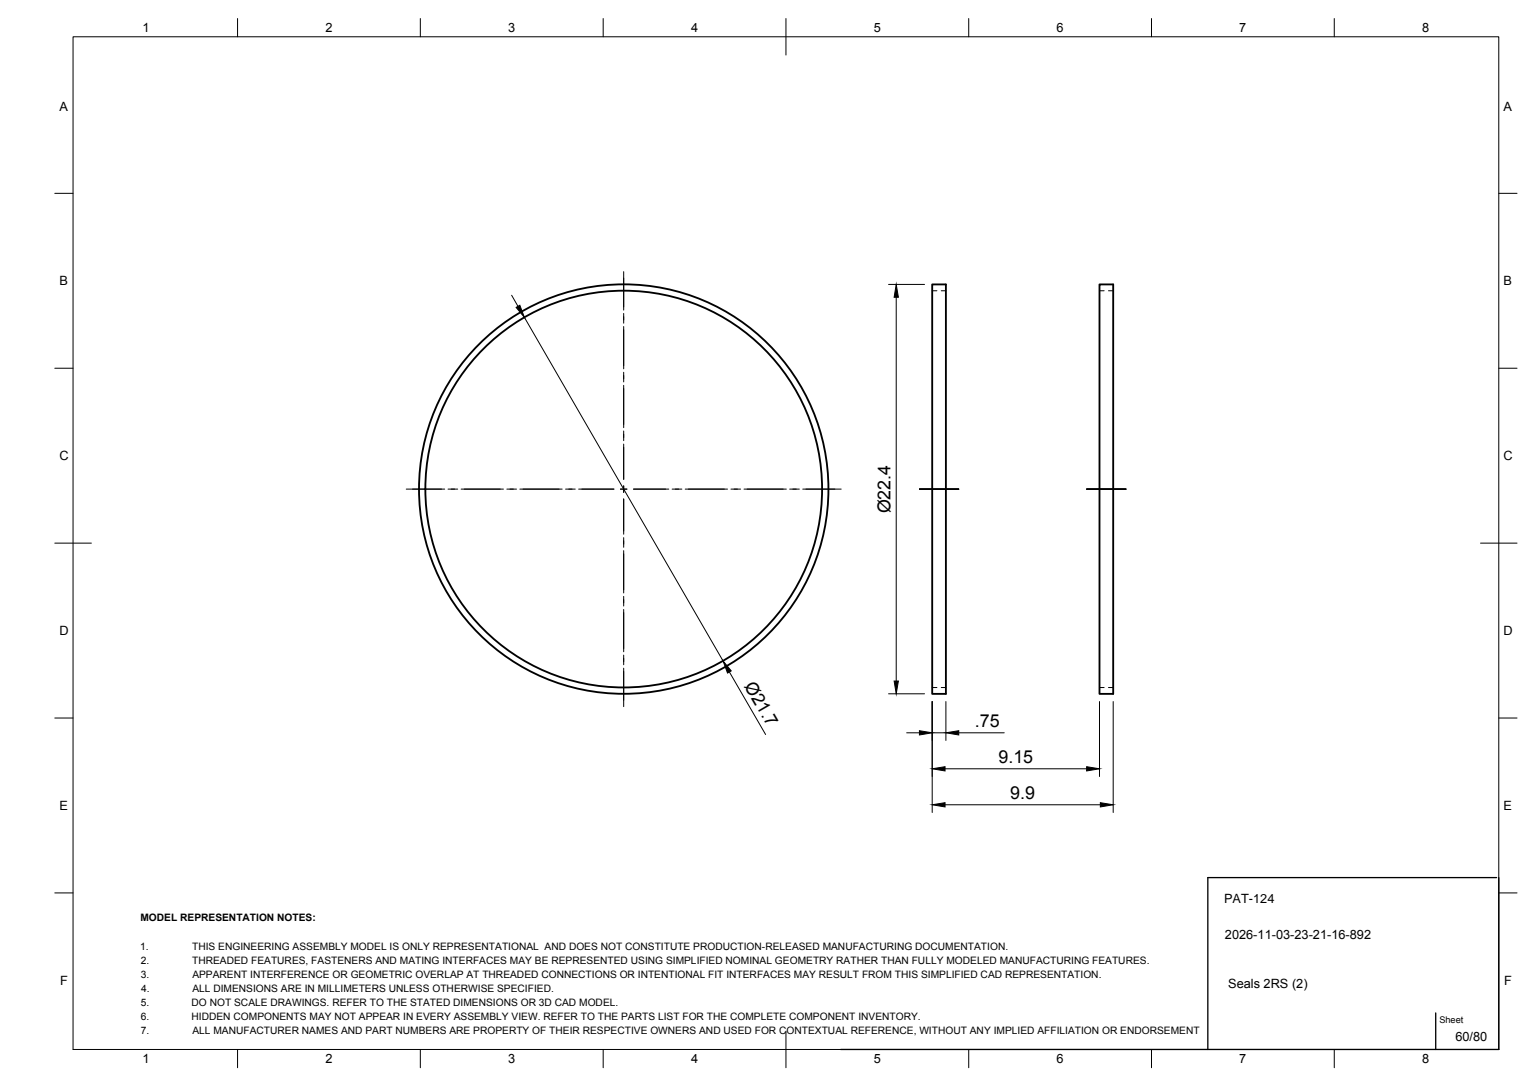
ISO-10303-21;
HEADER;
/* Generated by software containing ST-Developer
 * from STEP Tools, Inc. (www.steptools.com) 
 */

FILE_DESCRIPTION(
/* description */ ('XY cross-slide table'),
/* implementation_level */ '2;1');

FILE_NAME(
/* name */ 'Seals 2RS (2).step',
/* time_stamp */ '2026-10-28T03:22:46-07:00',
/* author */ (''),
/* organization */ (''),
/* preprocessor_version */ 'ST-DEVELOPER v20.2',
/* originating_system */ 'Autodesk Translation Framework v15.17.0.0',
/* authorisation */ '');

FILE_SCHEMA (('AUTOMOTIVE_DESIGN { 1 0 10303 214 3 1 1 }'));
ENDSEC;

DATA;
#10=MECHANICAL_DESIGN_GEOMETRIC_PRESENTATION_REPRESENTATION('',(#1746,#1747),#62984);
#1559=SHAPE_REPRESENTATION_RELATIONSHIP('SRR','None',#63415,#1642);
#1642=ADVANCED_BREP_SHAPE_REPRESENTATION('',(#1855,#1856),#62952);
#1746=STYLED_ITEM('',(#63912),#1855);
#1747=STYLED_ITEM('',(#63912),#1856);
#1855=MANIFOLD_SOLID_BREP('Body1',#23044);
#1856=MANIFOLD_SOLID_BREP('Body2',#23045);
#2206=FACE_BOUND('',#5349,.T.);
#2207=FACE_BOUND('',#5352,.T.);
#2208=FACE_BOUND('',#5355,.T.);
#2209=FACE_BOUND('',#5358,.T.);
#2674=PLANE('',#25637);
#2675=PLANE('',#25642);
#2676=PLANE('',#25645);
#2677=PLANE('',#25650);
#3715=FACE_OUTER_BOUND('',#5348,.T.);
#3716=FACE_OUTER_BOUND('',#5350,.T.);
#3717=FACE_OUTER_BOUND('',#5351,.T.);
#3718=FACE_OUTER_BOUND('',#5353,.T.);
#3719=FACE_OUTER_BOUND('',#5354,.T.);
#3720=FACE_OUTER_BOUND('',#5356,.T.);
#3721=FACE_OUTER_BOUND('',#5357,.T.);
#3722=FACE_OUTER_BOUND('',#5359,.T.);
#5348=EDGE_LOOP('',(#18802));
#5349=EDGE_LOOP('',(#18803));
#5350=EDGE_LOOP('',(#18804,#18805,#18806,#18807));
#5351=EDGE_LOOP('',(#18808));
#5352=EDGE_LOOP('',(#18809));
#5353=EDGE_LOOP('',(#18810,#18811,#18812,#18813));
#5354=EDGE_LOOP('',(#18814));
#5355=EDGE_LOOP('',(#18815));
#5356=EDGE_LOOP('',(#18816,#18817,#18818,#18819));
#5357=EDGE_LOOP('',(#18820));
#5358=EDGE_LOOP('',(#18821));
#5359=EDGE_LOOP('',(#18822,#18823,#18824,#18825));
#6849=LINE('',#49033,#8336);
#6850=LINE('',#49038,#8337);
#6851=LINE('',#49047,#8338);
#6852=LINE('',#49052,#8339);
#8336=VECTOR('',#30688,1.119765);
#8337=VECTOR('',#30695,1.085235);
#8338=VECTOR('',#30706,1.119765);
#8339=VECTOR('',#30713,1.085235);
#9528=CIRCLE('',#25638,1.119765);
#9529=CIRCLE('',#25639,1.085235);
#9530=CIRCLE('',#25641,1.119765);
#9531=CIRCLE('',#25643,1.085235);
#9532=CIRCLE('',#25646,1.119765);
#9533=CIRCLE('',#25647,1.085235);
#9534=CIRCLE('',#25649,1.119765);
#9535=CIRCLE('',#25651,1.085235);
#11087=VERTEX_POINT('',#49026);
#11088=VERTEX_POINT('',#49028);
#11089=VERTEX_POINT('',#49031);
#11090=VERTEX_POINT('',#49035);
#11091=VERTEX_POINT('',#49040);
#11092=VERTEX_POINT('',#49042);
#11093=VERTEX_POINT('',#49045);
#11094=VERTEX_POINT('',#49049);
#13785=EDGE_CURVE('',#11087,#11087,#9528,.T.);
#13786=EDGE_CURVE('',#11088,#11088,#9529,.T.);
#13787=EDGE_CURVE('',#11089,#11089,#9530,.T.);
#13788=EDGE_CURVE('',#11089,#11087,#6849,.T.);
#13789=EDGE_CURVE('',#11090,#11090,#9531,.T.);
#13790=EDGE_CURVE('',#11090,#11088,#6850,.T.);
#13791=EDGE_CURVE('',#11091,#11091,#9532,.T.);
#13792=EDGE_CURVE('',#11092,#11092,#9533,.T.);
#13793=EDGE_CURVE('',#11093,#11093,#9534,.T.);
#13794=EDGE_CURVE('',#11093,#11091,#6851,.T.);
#13795=EDGE_CURVE('',#11094,#11094,#9535,.T.);
#13796=EDGE_CURVE('',#11094,#11092,#6852,.T.);
#18802=ORIENTED_EDGE('',*,*,#13785,.F.);
#18803=ORIENTED_EDGE('',*,*,#13786,.T.);
#18804=ORIENTED_EDGE('',*,*,#13787,.F.);
#18805=ORIENTED_EDGE('',*,*,#13788,.T.);
#18806=ORIENTED_EDGE('',*,*,#13785,.T.);
#18807=ORIENTED_EDGE('',*,*,#13788,.F.);
#18808=ORIENTED_EDGE('',*,*,#13787,.T.);
#18809=ORIENTED_EDGE('',*,*,#13789,.F.);
#18810=ORIENTED_EDGE('',*,*,#13789,.T.);
#18811=ORIENTED_EDGE('',*,*,#13790,.T.);
#18812=ORIENTED_EDGE('',*,*,#13786,.F.);
#18813=ORIENTED_EDGE('',*,*,#13790,.F.);
#18814=ORIENTED_EDGE('',*,*,#13791,.F.);
#18815=ORIENTED_EDGE('',*,*,#13792,.T.);
#18816=ORIENTED_EDGE('',*,*,#13793,.F.);
#18817=ORIENTED_EDGE('',*,*,#13794,.T.);
#18818=ORIENTED_EDGE('',*,*,#13791,.T.);
#18819=ORIENTED_EDGE('',*,*,#13794,.F.);
#18820=ORIENTED_EDGE('',*,*,#13793,.T.);
#18821=ORIENTED_EDGE('',*,*,#13795,.F.);
#18822=ORIENTED_EDGE('',*,*,#13795,.T.);
#18823=ORIENTED_EDGE('',*,*,#13796,.T.);
#18824=ORIENTED_EDGE('',*,*,#13792,.F.);
#18825=ORIENTED_EDGE('',*,*,#13796,.F.);
#21424=CYLINDRICAL_SURFACE('',#25640,1.119765);
#21425=CYLINDRICAL_SURFACE('',#25644,1.085235);
#21426=CYLINDRICAL_SURFACE('',#25648,1.119765);
#21427=CYLINDRICAL_SURFACE('',#25652,1.085235);
#22496=ADVANCED_FACE('',(#3715,#2206),#2674,.T.);
#22497=ADVANCED_FACE('',(#3716),#21424,.T.);
#22498=ADVANCED_FACE('',(#3717,#2207),#2675,.T.);
#22499=ADVANCED_FACE('',(#3718),#21425,.F.);
#22500=ADVANCED_FACE('',(#3719,#2208),#2676,.T.);
#22501=ADVANCED_FACE('',(#3720),#21426,.T.);
#22502=ADVANCED_FACE('',(#3721,#2209),#2677,.T.);
#22503=ADVANCED_FACE('',(#3722),#21427,.F.);
#23044=CLOSED_SHELL('',(#22496,#22497,#22498,#22499));
#23045=CLOSED_SHELL('',(#22500,#22501,#22502,#22503));
#25636=AXIS2_PLACEMENT_3D('',#49024,#30676,#30677);
#25637=AXIS2_PLACEMENT_3D('',#49025,#30678,#30679);
#25638=AXIS2_PLACEMENT_3D('',#49027,#30680,#30681);
#25639=AXIS2_PLACEMENT_3D('',#49029,#30682,#30683);
#25640=AXIS2_PLACEMENT_3D('',#49030,#30684,#30685);
#25641=AXIS2_PLACEMENT_3D('',#49032,#30686,#30687);
#25642=AXIS2_PLACEMENT_3D('',#49034,#30689,#30690);
#25643=AXIS2_PLACEMENT_3D('',#49036,#30691,#30692);
#25644=AXIS2_PLACEMENT_3D('',#49037,#30693,#30694);
#25645=AXIS2_PLACEMENT_3D('',#49039,#30696,#30697);
#25646=AXIS2_PLACEMENT_3D('',#49041,#30698,#30699);
#25647=AXIS2_PLACEMENT_3D('',#49043,#30700,#30701);
#25648=AXIS2_PLACEMENT_3D('',#49044,#30702,#30703);
#25649=AXIS2_PLACEMENT_3D('',#49046,#30704,#30705);
#25650=AXIS2_PLACEMENT_3D('',#49048,#30707,#30708);
#25651=AXIS2_PLACEMENT_3D('',#49050,#30709,#30710);
#25652=AXIS2_PLACEMENT_3D('',#49051,#30711,#30712);
#30676=DIRECTION('axis',(0.,0.,1.));
#30677=DIRECTION('refdir',(1.,0.,0.));
#30678=DIRECTION('center_axis',(0.,1.,0.));
#30679=DIRECTION('ref_axis',(0.,0.,1.));
#30680=DIRECTION('center_axis',(0.,-1.,0.));
#30681=DIRECTION('ref_axis',(1.,0.,0.));
#30682=DIRECTION('center_axis',(0.,-1.,0.));
#30683=DIRECTION('ref_axis',(1.,0.,0.));
#30684=DIRECTION('center_axis',(0.,-1.,0.));
#30685=DIRECTION('ref_axis',(1.,0.,0.));
#30686=DIRECTION('center_axis',(0.,-1.,0.));
#30687=DIRECTION('ref_axis',(1.,0.,0.));
#30688=DIRECTION('',(0.,1.,0.));
#30689=DIRECTION('center_axis',(0.,-1.,0.));
#30690=DIRECTION('ref_axis',(0.,0.,-1.));
#30691=DIRECTION('center_axis',(0.,-1.,0.));
#30692=DIRECTION('ref_axis',(1.,0.,0.));
#30693=DIRECTION('center_axis',(0.,-1.,0.));
#30694=DIRECTION('ref_axis',(1.,0.,0.));
#30695=DIRECTION('',(0.,1.,0.));
#30696=DIRECTION('center_axis',(0.,1.,0.));
#30697=DIRECTION('ref_axis',(0.,0.,1.));
#30698=DIRECTION('center_axis',(0.,-1.,0.));
#30699=DIRECTION('ref_axis',(1.,0.,0.));
#30700=DIRECTION('center_axis',(0.,-1.,0.));
#30701=DIRECTION('ref_axis',(1.,0.,0.));
#30702=DIRECTION('center_axis',(0.,-1.,0.));
#30703=DIRECTION('ref_axis',(1.,0.,0.));
#30704=DIRECTION('center_axis',(0.,-1.,0.));
#30705=DIRECTION('ref_axis',(1.,0.,0.));
#30706=DIRECTION('',(0.,1.,0.));
#30707=DIRECTION('center_axis',(0.,-1.,0.));
#30708=DIRECTION('ref_axis',(0.,0.,-1.));
#30709=DIRECTION('center_axis',(0.,-1.,0.));
#30710=DIRECTION('ref_axis',(1.,0.,0.));
#30711=DIRECTION('center_axis',(0.,-1.,0.));
#30712=DIRECTION('ref_axis',(1.,0.,0.));
#30713=DIRECTION('',(0.,1.,0.));
#49024=CARTESIAN_POINT('',(0.,0.,0.));
#49025=CARTESIAN_POINT('Origin',(1.119765,0.495,0.));
#49026=CARTESIAN_POINT('',(-1.119765,0.495,-1.37131662304724E-16));
#49027=CARTESIAN_POINT('Origin',(0.,0.495,0.));
#49028=CARTESIAN_POINT('',(-1.085235,0.495,-1.32902956907268E-16));
#49029=CARTESIAN_POINT('Origin',(0.,0.495,0.));
#49030=CARTESIAN_POINT('Origin',(0.,0.4575,0.));
#49031=CARTESIAN_POINT('',(-1.119765,0.42,-1.37131662304724E-16));
#49032=CARTESIAN_POINT('Origin',(0.,0.42,0.));
#49033=CARTESIAN_POINT('',(-1.119765,0.4575,-1.37131662304724E-16));
#49034=CARTESIAN_POINT('Origin',(1.085235,0.42,0.));
#49035=CARTESIAN_POINT('',(-1.085235,0.42,-1.32902956907268E-16));
#49036=CARTESIAN_POINT('Origin',(0.,0.42,0.));
#49037=CARTESIAN_POINT('Origin',(0.,0.4575,0.));
#49038=CARTESIAN_POINT('',(-1.085235,0.4575,-1.32902956907268E-16));
#49039=CARTESIAN_POINT('Origin',(1.119765,-0.42,0.));
#49040=CARTESIAN_POINT('',(-1.119765,-0.42,-1.37131662304724E-16));
#49041=CARTESIAN_POINT('Origin',(0.,-0.42,0.));
#49042=CARTESIAN_POINT('',(-1.085235,-0.42,-1.32902956907268E-16));
#49043=CARTESIAN_POINT('Origin',(0.,-0.42,0.));
#49044=CARTESIAN_POINT('Origin',(0.,-0.4575,0.));
#49045=CARTESIAN_POINT('',(-1.119765,-0.495,-1.37131662304724E-16));
#49046=CARTESIAN_POINT('Origin',(0.,-0.495,0.));
#49047=CARTESIAN_POINT('',(-1.119765,-0.4575,-1.37131662304724E-16));
#49048=CARTESIAN_POINT('Origin',(1.085235,-0.495,0.));
#49049=CARTESIAN_POINT('',(-1.085235,-0.495,-1.32902956907268E-16));
#49050=CARTESIAN_POINT('Origin',(0.,-0.495,0.));
#49051=CARTESIAN_POINT('Origin',(0.,-0.4575,0.));
#49052=CARTESIAN_POINT('',(-1.085235,-0.4575,-1.32902956907268E-16));
#62853=UNCERTAINTY_MEASURE_WITH_UNIT(LENGTH_MEASURE(0.001),#62985,
'DISTANCE_ACCURACY_VALUE',
'Maximum model space distance between geometric entities at asserted c
onnectivities');
#62885=UNCERTAINTY_MEASURE_WITH_UNIT(LENGTH_MEASURE(0.001),#62985,
'DISTANCE_ACCURACY_VALUE',
'Maximum model space distance between geometric entities at asserted c
onnectivities');
#62952=(
GEOMETRIC_REPRESENTATION_CONTEXT(3)
GLOBAL_UNCERTAINTY_ASSIGNED_CONTEXT((#62853))
GLOBAL_UNIT_ASSIGNED_CONTEXT((#62985,#62987,#62988))
REPRESENTATION_CONTEXT('','3D')
);
#62984=(
GEOMETRIC_REPRESENTATION_CONTEXT(3)
GLOBAL_UNCERTAINTY_ASSIGNED_CONTEXT((#62885))
GLOBAL_UNIT_ASSIGNED_CONTEXT((#62985,#62987,#62988))
REPRESENTATION_CONTEXT('','3D')
);
#62985=(
LENGTH_UNIT()
NAMED_UNIT(*)
SI_UNIT(.CENTI.,.METRE.)
);
#62987=(
NAMED_UNIT(*)
PLANE_ANGLE_UNIT()
SI_UNIT($,.RADIAN.)
);
#62988=(
NAMED_UNIT(*)
SI_UNIT($,.STERADIAN.)
SOLID_ANGLE_UNIT()
);
#63055=SHAPE_DEFINITION_REPRESENTATION(#63233,#63415);
#63233=PRODUCT_DEFINITION_SHAPE('',$,#63514);
#63415=SHAPE_REPRESENTATION('',(#25636),#62952);
#63447=PRODUCT_DEFINITION_CONTEXT('part definition',#63743,'design');
#63514=PRODUCT_DEFINITION('Seals 2RS (2)','Seals 2RS (2)',#63612,#63447);
#63612=PRODUCT_DEFINITION_FORMATION('',$,#63811);
#63743=APPLICATION_CONTEXT(
'Core Data for Automotive Mechanical Design Process');
#63744=PRODUCT_CONTEXT('part definition',#63743,'mechanical');
#63811=PRODUCT('Seals 2RS (2)','Seals 2RS (2)','Seals 2RS (2)',(#63744));
#63906=COLOUR_RGB('Grey',0.48,0.52,0.57);
#63907=FILL_AREA_STYLE_COLOUR('',#63906);
#63908=FILL_AREA_STYLE('',(#63907));
#63909=SURFACE_STYLE_FILL_AREA(#63908);
#63910=SURFACE_SIDE_STYLE('',(#63909));
#63911=SURFACE_STYLE_USAGE(.BOTH.,#63910);
#63912=PRESENTATION_STYLE_ASSIGNMENT((#63911));
ENDSEC;
END-ISO-10303-21;
